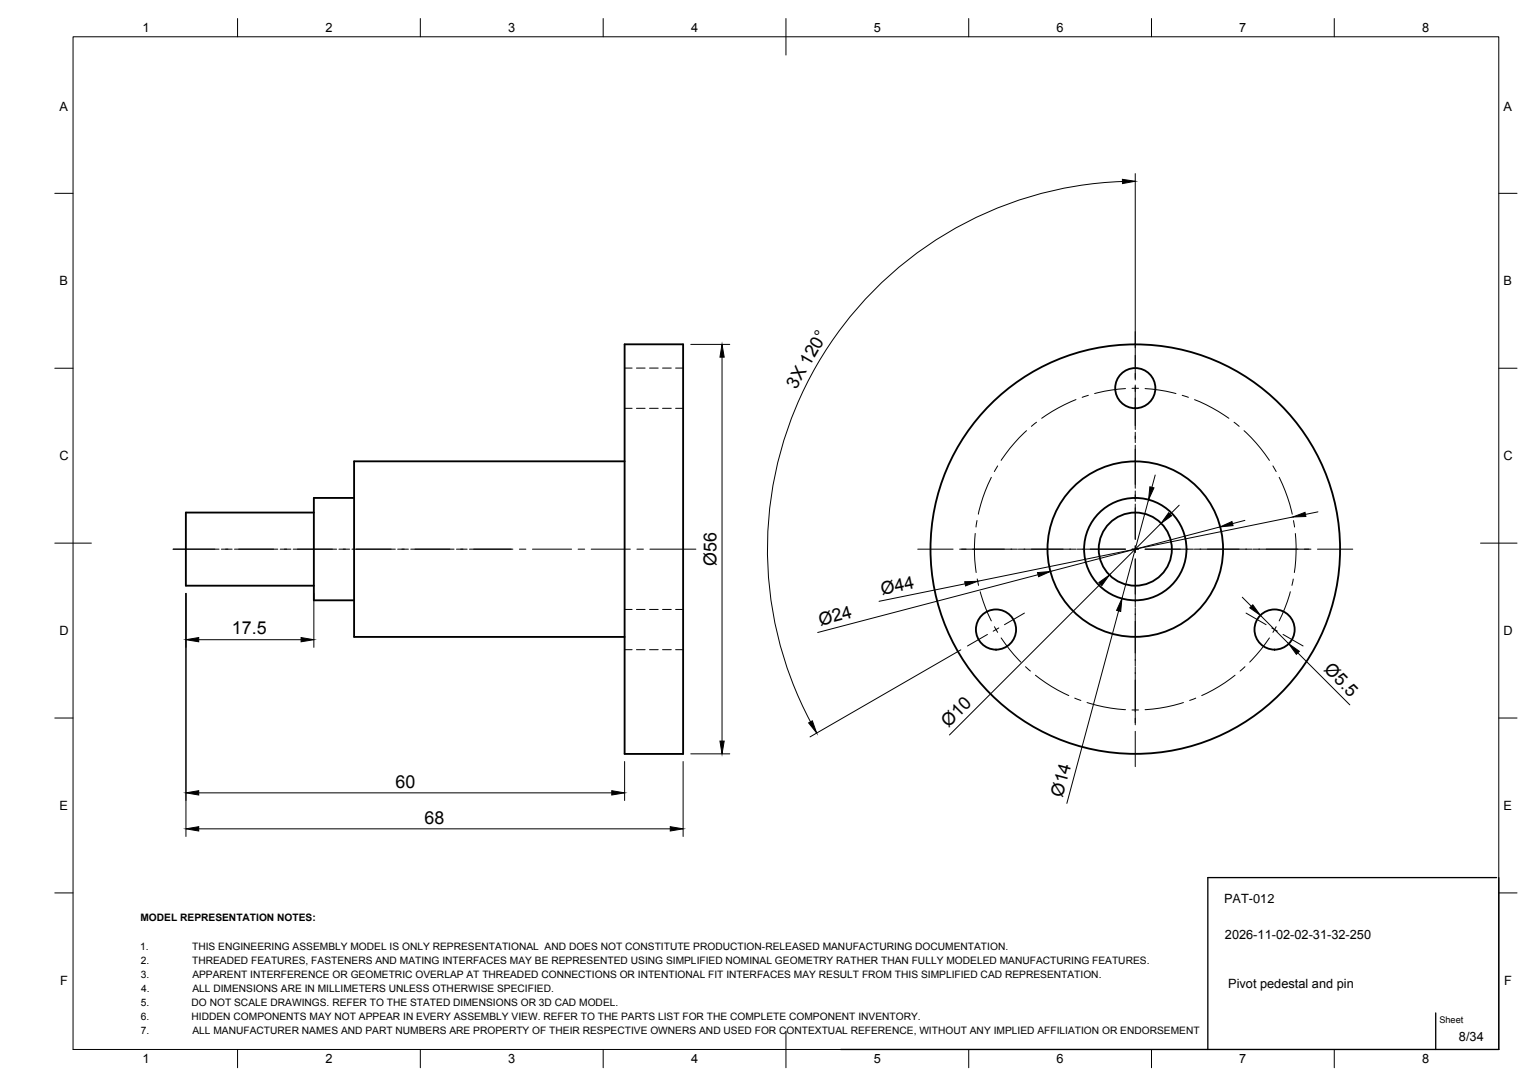
ISO-10303-21;
HEADER;
/* Generated by software containing ST-Developer
 * from STEP Tools, Inc. (www.steptools.com) 
 */

FILE_DESCRIPTION(
/* description */ ('Belt tensioner idler arm'),
/* implementation_level */ '2;1');

FILE_NAME(
/* name */ 'Pivot pedestal and pin.step',
/* time_stamp */ '2026-10-28T03:22:15-07:00',
/* author */ (''),
/* organization */ (''),
/* preprocessor_version */ 'ST-DEVELOPER v20.2',
/* originating_system */ 'Autodesk Translation Framework v15.17.0.0',
/* authorisation */ '');

FILE_SCHEMA (('AUTOMOTIVE_DESIGN { 1 0 10303 214 3 1 1 }'));
ENDSEC;

DATA;
#10=MECHANICAL_DESIGN_GEOMETRIC_PRESENTATION_REPRESENTATION('',(#450),#12779);
#382=SHAPE_REPRESENTATION_RELATIONSHIP('SRR','None',#12928,#416);
#416=ADVANCED_BREP_SHAPE_REPRESENTATION('',(#492),#12745);
#450=STYLED_ITEM('',(#13184),#492);
#492=MANIFOLD_SOLID_BREP('Body1',#6184);
#537=FACE_BOUND('',#1241,.T.);
#538=FACE_BOUND('',#1246,.T.);
#539=FACE_BOUND('',#1247,.T.);
#540=FACE_BOUND('',#1248,.T.);
#541=FACE_BOUND('',#1249,.T.);
#542=FACE_BOUND('',#1253,.T.);
#543=FACE_BOUND('',#1255,.T.);
#544=FACE_BOUND('',#1256,.T.);
#545=FACE_BOUND('',#1257,.T.);
#681=PLANE('',#6650);
#682=PLANE('',#6657);
#683=PLANE('',#6658);
#684=PLANE('',#6665);
#685=PLANE('',#6666);
#860=FACE_OUTER_BOUND('',#1237,.T.);
#861=FACE_OUTER_BOUND('',#1238,.T.);
#862=FACE_OUTER_BOUND('',#1239,.T.);
#863=FACE_OUTER_BOUND('',#1240,.T.);
#864=FACE_OUTER_BOUND('',#1242,.T.);
#865=FACE_OUTER_BOUND('',#1243,.T.);
#866=FACE_OUTER_BOUND('',#1244,.T.);
#867=FACE_OUTER_BOUND('',#1245,.T.);
#868=FACE_OUTER_BOUND('',#1250,.T.);
#869=FACE_OUTER_BOUND('',#1251,.T.);
#870=FACE_OUTER_BOUND('',#1252,.T.);
#871=FACE_OUTER_BOUND('',#1254,.T.);
#1237=EDGE_LOOP('',(#4188,#4189,#4190,#4191));
#1238=EDGE_LOOP('',(#4192,#4193,#4194,#4195));
#1239=EDGE_LOOP('',(#4196,#4197,#4198,#4199));
#1240=EDGE_LOOP('',(#4200));
#1241=EDGE_LOOP('',(#4201));
#1242=EDGE_LOOP('',(#4202,#4203,#4204,#4205));
#1243=EDGE_LOOP('',(#4206,#4207,#4208,#4209));
#1244=EDGE_LOOP('',(#4210));
#1245=EDGE_LOOP('',(#4211));
#1246=EDGE_LOOP('',(#4212));
#1247=EDGE_LOOP('',(#4213));
#1248=EDGE_LOOP('',(#4214));
#1249=EDGE_LOOP('',(#4215));
#1250=EDGE_LOOP('',(#4216,#4217,#4218,#4219));
#1251=EDGE_LOOP('',(#4220,#4221,#4222,#4223));
#1252=EDGE_LOOP('',(#4224));
#1253=EDGE_LOOP('',(#4225));
#1254=EDGE_LOOP('',(#4226));
#1255=EDGE_LOOP('',(#4227));
#1256=EDGE_LOOP('',(#4228));
#1257=EDGE_LOOP('',(#4229));
#1748=LINE('',#9562,#2097);
#1749=LINE('',#9568,#2098);
#1750=LINE('',#9574,#2099);
#1751=LINE('',#9583,#2100);
#1752=LINE('',#9588,#2101);
#1753=LINE('',#9597,#2102);
#1754=LINE('',#9602,#2103);
#2097=VECTOR('',#7556,0.275);
#2098=VECTOR('',#7563,0.275);
#2099=VECTOR('',#7570,0.275);
#2100=VECTOR('',#7581,0.7);
#2101=VECTOR('',#7588,0.5);
#2102=VECTOR('',#7599,2.8);
#2103=VECTOR('',#7606,1.2);
#2415=CIRCLE('',#6642,0.275);
#2416=CIRCLE('',#6643,0.275);
#2417=CIRCLE('',#6645,0.275);
#2418=CIRCLE('',#6646,0.275);
#2419=CIRCLE('',#6648,0.275);
#2420=CIRCLE('',#6649,0.275);
#2421=CIRCLE('',#6651,0.7);
#2422=CIRCLE('',#6652,0.5);
#2423=CIRCLE('',#6654,0.7);
#2424=CIRCLE('',#6656,0.5);
#2425=CIRCLE('',#6659,2.8);
#2426=CIRCLE('',#6660,1.2);
#2427=CIRCLE('',#6662,2.8);
#2428=CIRCLE('',#6664,1.2);
#2803=VERTEX_POINT('',#9559);
#2804=VERTEX_POINT('',#9561);
#2805=VERTEX_POINT('',#9565);
#2806=VERTEX_POINT('',#9567);
#2807=VERTEX_POINT('',#9571);
#2808=VERTEX_POINT('',#9573);
#2809=VERTEX_POINT('',#9577);
#2810=VERTEX_POINT('',#9579);
#2811=VERTEX_POINT('',#9582);
#2812=VERTEX_POINT('',#9586);
#2813=VERTEX_POINT('',#9591);
#2814=VERTEX_POINT('',#9593);
#2815=VERTEX_POINT('',#9596);
#2816=VERTEX_POINT('',#9600);
#3349=EDGE_CURVE('',#2803,#2803,#2415,.T.);
#3350=EDGE_CURVE('',#2803,#2804,#1748,.T.);
#3351=EDGE_CURVE('',#2804,#2804,#2416,.T.);
#3352=EDGE_CURVE('',#2805,#2805,#2417,.T.);
#3353=EDGE_CURVE('',#2805,#2806,#1749,.T.);
#3354=EDGE_CURVE('',#2806,#2806,#2418,.T.);
#3355=EDGE_CURVE('',#2807,#2807,#2419,.T.);
#3356=EDGE_CURVE('',#2807,#2808,#1750,.T.);
#3357=EDGE_CURVE('',#2808,#2808,#2420,.T.);
#3358=EDGE_CURVE('',#2809,#2809,#2421,.T.);
#3359=EDGE_CURVE('',#2810,#2810,#2422,.T.);
#3360=EDGE_CURVE('',#2809,#2811,#1751,.T.);
#3361=EDGE_CURVE('',#2811,#2811,#2423,.T.);
#3362=EDGE_CURVE('',#2812,#2812,#2424,.T.);
#3363=EDGE_CURVE('',#2812,#2810,#1752,.T.);
#3364=EDGE_CURVE('',#2813,#2813,#2425,.T.);
#3365=EDGE_CURVE('',#2814,#2814,#2426,.T.);
#3366=EDGE_CURVE('',#2813,#2815,#1753,.T.);
#3367=EDGE_CURVE('',#2815,#2815,#2427,.T.);
#3368=EDGE_CURVE('',#2816,#2816,#2428,.T.);
#3369=EDGE_CURVE('',#2816,#2814,#1754,.T.);
#4188=ORIENTED_EDGE('',*,*,#3349,.F.);
#4189=ORIENTED_EDGE('',*,*,#3350,.T.);
#4190=ORIENTED_EDGE('',*,*,#3351,.F.);
#4191=ORIENTED_EDGE('',*,*,#3350,.F.);
#4192=ORIENTED_EDGE('',*,*,#3352,.F.);
#4193=ORIENTED_EDGE('',*,*,#3353,.T.);
#4194=ORIENTED_EDGE('',*,*,#3354,.F.);
#4195=ORIENTED_EDGE('',*,*,#3353,.F.);
#4196=ORIENTED_EDGE('',*,*,#3355,.F.);
#4197=ORIENTED_EDGE('',*,*,#3356,.T.);
#4198=ORIENTED_EDGE('',*,*,#3357,.F.);
#4199=ORIENTED_EDGE('',*,*,#3356,.F.);
#4200=ORIENTED_EDGE('',*,*,#3358,.T.);
#4201=ORIENTED_EDGE('',*,*,#3359,.F.);
#4202=ORIENTED_EDGE('',*,*,#3358,.F.);
#4203=ORIENTED_EDGE('',*,*,#3360,.T.);
#4204=ORIENTED_EDGE('',*,*,#3361,.F.);
#4205=ORIENTED_EDGE('',*,*,#3360,.F.);
#4206=ORIENTED_EDGE('',*,*,#3362,.F.);
#4207=ORIENTED_EDGE('',*,*,#3363,.T.);
#4208=ORIENTED_EDGE('',*,*,#3359,.T.);
#4209=ORIENTED_EDGE('',*,*,#3363,.F.);
#4210=ORIENTED_EDGE('',*,*,#3362,.T.);
#4211=ORIENTED_EDGE('',*,*,#3364,.T.);
#4212=ORIENTED_EDGE('',*,*,#3351,.T.);
#4213=ORIENTED_EDGE('',*,*,#3354,.T.);
#4214=ORIENTED_EDGE('',*,*,#3357,.T.);
#4215=ORIENTED_EDGE('',*,*,#3365,.F.);
#4216=ORIENTED_EDGE('',*,*,#3364,.F.);
#4217=ORIENTED_EDGE('',*,*,#3366,.T.);
#4218=ORIENTED_EDGE('',*,*,#3367,.T.);
#4219=ORIENTED_EDGE('',*,*,#3366,.F.);
#4220=ORIENTED_EDGE('',*,*,#3368,.F.);
#4221=ORIENTED_EDGE('',*,*,#3369,.T.);
#4222=ORIENTED_EDGE('',*,*,#3365,.T.);
#4223=ORIENTED_EDGE('',*,*,#3369,.F.);
#4224=ORIENTED_EDGE('',*,*,#3368,.T.);
#4225=ORIENTED_EDGE('',*,*,#3361,.T.);
#4226=ORIENTED_EDGE('',*,*,#3367,.F.);
#4227=ORIENTED_EDGE('',*,*,#3349,.T.);
#4228=ORIENTED_EDGE('',*,*,#3352,.T.);
#4229=ORIENTED_EDGE('',*,*,#3355,.T.);
#5667=CYLINDRICAL_SURFACE('',#6641,0.275);
#5668=CYLINDRICAL_SURFACE('',#6644,0.275);
#5669=CYLINDRICAL_SURFACE('',#6647,0.275);
#5670=CYLINDRICAL_SURFACE('',#6653,0.7);
#5671=CYLINDRICAL_SURFACE('',#6655,0.5);
#5672=CYLINDRICAL_SURFACE('',#6661,2.8);
#5673=CYLINDRICAL_SURFACE('',#6663,1.2);
#5837=ADVANCED_FACE('',(#860),#5667,.F.);
#5838=ADVANCED_FACE('',(#861),#5668,.F.);
#5839=ADVANCED_FACE('',(#862),#5669,.F.);
#5840=ADVANCED_FACE('',(#863,#537),#681,.T.);
#5841=ADVANCED_FACE('',(#864),#5670,.T.);
#5842=ADVANCED_FACE('',(#865),#5671,.T.);
#5843=ADVANCED_FACE('',(#866),#682,.T.);
#5844=ADVANCED_FACE('',(#867,#538,#539,#540,#541),#683,.T.);
#5845=ADVANCED_FACE('',(#868),#5672,.T.);
#5846=ADVANCED_FACE('',(#869),#5673,.T.);
#5847=ADVANCED_FACE('',(#870,#542),#684,.T.);
#5848=ADVANCED_FACE('',(#871,#543,#544,#545),#685,.F.);
#6184=CLOSED_SHELL('',(#5837,#5838,#5839,#5840,#5841,#5842,#5843,#5844,
#5845,#5846,#5847,#5848));
#6640=AXIS2_PLACEMENT_3D('',#9557,#7550,#7551);
#6641=AXIS2_PLACEMENT_3D('',#9558,#7552,#7553);
#6642=AXIS2_PLACEMENT_3D('',#9560,#7554,#7555);
#6643=AXIS2_PLACEMENT_3D('',#9563,#7557,#7558);
#6644=AXIS2_PLACEMENT_3D('',#9564,#7559,#7560);
#6645=AXIS2_PLACEMENT_3D('',#9566,#7561,#7562);
#6646=AXIS2_PLACEMENT_3D('',#9569,#7564,#7565);
#6647=AXIS2_PLACEMENT_3D('',#9570,#7566,#7567);
#6648=AXIS2_PLACEMENT_3D('',#9572,#7568,#7569);
#6649=AXIS2_PLACEMENT_3D('',#9575,#7571,#7572);
#6650=AXIS2_PLACEMENT_3D('',#9576,#7573,#7574);
#6651=AXIS2_PLACEMENT_3D('',#9578,#7575,#7576);
#6652=AXIS2_PLACEMENT_3D('',#9580,#7577,#7578);
#6653=AXIS2_PLACEMENT_3D('',#9581,#7579,#7580);
#6654=AXIS2_PLACEMENT_3D('',#9584,#7582,#7583);
#6655=AXIS2_PLACEMENT_3D('',#9585,#7584,#7585);
#6656=AXIS2_PLACEMENT_3D('',#9587,#7586,#7587);
#6657=AXIS2_PLACEMENT_3D('',#9589,#7589,#7590);
#6658=AXIS2_PLACEMENT_3D('',#9590,#7591,#7592);
#6659=AXIS2_PLACEMENT_3D('',#9592,#7593,#7594);
#6660=AXIS2_PLACEMENT_3D('',#9594,#7595,#7596);
#6661=AXIS2_PLACEMENT_3D('',#9595,#7597,#7598);
#6662=AXIS2_PLACEMENT_3D('',#9598,#7600,#7601);
#6663=AXIS2_PLACEMENT_3D('',#9599,#7602,#7603);
#6664=AXIS2_PLACEMENT_3D('',#9601,#7604,#7605);
#6665=AXIS2_PLACEMENT_3D('',#9603,#7607,#7608);
#6666=AXIS2_PLACEMENT_3D('',#9604,#7609,#7610);
#7550=DIRECTION('axis',(0.,0.,1.));
#7551=DIRECTION('refdir',(1.,0.,0.));
#7552=DIRECTION('center_axis',(0.,0.,1.));
#7553=DIRECTION('ref_axis',(1.,0.,0.));
#7554=DIRECTION('center_axis',(0.,0.,1.));
#7555=DIRECTION('ref_axis',(1.,0.,0.));
#7556=DIRECTION('',(0.,0.,1.));
#7557=DIRECTION('center_axis',(0.,0.,-1.));
#7558=DIRECTION('ref_axis',(1.,0.,0.));
#7559=DIRECTION('center_axis',(0.,0.,1.));
#7560=DIRECTION('ref_axis',(1.,0.,0.));
#7561=DIRECTION('center_axis',(0.,0.,1.));
#7562=DIRECTION('ref_axis',(1.,0.,0.));
#7563=DIRECTION('',(0.,0.,1.));
#7564=DIRECTION('center_axis',(0.,0.,-1.));
#7565=DIRECTION('ref_axis',(1.,0.,0.));
#7566=DIRECTION('center_axis',(0.,0.,1.));
#7567=DIRECTION('ref_axis',(1.,0.,0.));
#7568=DIRECTION('center_axis',(0.,0.,1.));
#7569=DIRECTION('ref_axis',(1.,0.,0.));
#7570=DIRECTION('',(0.,0.,1.));
#7571=DIRECTION('center_axis',(0.,0.,-1.));
#7572=DIRECTION('ref_axis',(1.,0.,0.));
#7573=DIRECTION('center_axis',(0.,0.,1.));
#7574=DIRECTION('ref_axis',(1.,0.,0.));
#7575=DIRECTION('center_axis',(0.,0.,1.));
#7576=DIRECTION('ref_axis',(1.,0.,0.));
#7577=DIRECTION('center_axis',(0.,0.,1.));
#7578=DIRECTION('ref_axis',(1.,0.,0.));
#7579=DIRECTION('center_axis',(0.,0.,1.));
#7580=DIRECTION('ref_axis',(1.,0.,0.));
#7581=DIRECTION('',(0.,0.,-1.));
#7582=DIRECTION('center_axis',(0.,0.,-1.));
#7583=DIRECTION('ref_axis',(1.,0.,0.));
#7584=DIRECTION('center_axis',(0.,0.,1.));
#7585=DIRECTION('ref_axis',(1.,0.,0.));
#7586=DIRECTION('center_axis',(0.,0.,1.));
#7587=DIRECTION('ref_axis',(1.,0.,0.));
#7588=DIRECTION('',(0.,0.,-1.));
#7589=DIRECTION('center_axis',(0.,0.,1.));
#7590=DIRECTION('ref_axis',(1.,0.,0.));
#7591=DIRECTION('center_axis',(0.,0.,1.));
#7592=DIRECTION('ref_axis',(1.,0.,0.));
#7593=DIRECTION('center_axis',(0.,0.,1.));
#7594=DIRECTION('ref_axis',(1.,0.,0.));
#7595=DIRECTION('center_axis',(0.,0.,1.));
#7596=DIRECTION('ref_axis',(1.,0.,0.));
#7597=DIRECTION('center_axis',(0.,0.,1.));
#7598=DIRECTION('ref_axis',(1.,0.,0.));
#7599=DIRECTION('',(0.,0.,-1.));
#7600=DIRECTION('center_axis',(0.,0.,1.));
#7601=DIRECTION('ref_axis',(1.,0.,0.));
#7602=DIRECTION('center_axis',(0.,0.,1.));
#7603=DIRECTION('ref_axis',(1.,0.,0.));
#7604=DIRECTION('center_axis',(0.,0.,1.));
#7605=DIRECTION('ref_axis',(1.,0.,0.));
#7606=DIRECTION('',(0.,0.,-1.));
#7607=DIRECTION('center_axis',(0.,0.,1.));
#7608=DIRECTION('ref_axis',(1.,0.,0.));
#7609=DIRECTION('center_axis',(0.,0.,1.));
#7610=DIRECTION('ref_axis',(1.,0.,0.));
#9557=CARTESIAN_POINT('',(0.,0.,0.));
#9558=CARTESIAN_POINT('Origin',(2.2,0.,-0.1));
#9559=CARTESIAN_POINT('',(1.925,-3.36777869765522E-17,0.));
#9560=CARTESIAN_POINT('Origin',(2.2,0.,0.));
#9561=CARTESIAN_POINT('',(1.925,3.36777869765522E-17,0.8));
#9562=CARTESIAN_POINT('',(1.925,-3.36777869765522E-17,-0.1));
#9563=CARTESIAN_POINT('Origin',(2.2,0.,0.8));
#9564=CARTESIAN_POINT('Origin',(-1.1,1.90525588832577,-0.1));
#9565=CARTESIAN_POINT('',(-1.375,1.90525588832577,0.));
#9566=CARTESIAN_POINT('Origin',(-1.1,1.90525588832577,0.));
#9567=CARTESIAN_POINT('',(-1.375,1.90525588832577,0.8));
#9568=CARTESIAN_POINT('',(-1.375,1.90525588832577,-0.1));
#9569=CARTESIAN_POINT('Origin',(-1.1,1.90525588832577,0.8));
#9570=CARTESIAN_POINT('Origin',(-1.1,-1.90525588832576,-0.1));
#9571=CARTESIAN_POINT('',(-1.375,-1.90525588832576,0.));
#9572=CARTESIAN_POINT('Origin',(-1.1,-1.90525588832576,0.));
#9573=CARTESIAN_POINT('',(-1.375,-1.90525588832576,0.8));
#9574=CARTESIAN_POINT('',(-1.375,-1.90525588832576,-0.1));
#9575=CARTESIAN_POINT('Origin',(-1.1,-1.90525588832576,0.8));
#9576=CARTESIAN_POINT('Origin',(0.,0.,5.05));
#9577=CARTESIAN_POINT('',(-0.7,-8.57252759403147E-17,5.05));
#9578=CARTESIAN_POINT('Origin',(0.,0.,5.05));
#9579=CARTESIAN_POINT('',(-0.5,-6.12323399573677E-17,5.05));
#9580=CARTESIAN_POINT('Origin',(0.,0.,5.05));
#9581=CARTESIAN_POINT('Origin',(0.,0.,4.5));
#9582=CARTESIAN_POINT('',(-0.7,-8.57252759403147E-17,4.5));
#9583=CARTESIAN_POINT('',(-0.7,-8.57252759403147E-17,4.5));
#9584=CARTESIAN_POINT('Origin',(0.,0.,4.5));
#9585=CARTESIAN_POINT('Origin',(0.,0.,4.5));
#9586=CARTESIAN_POINT('',(-0.5,-6.12323399573677E-17,6.8));
#9587=CARTESIAN_POINT('Origin',(0.,0.,6.8));
#9588=CARTESIAN_POINT('',(-0.5,-6.12323399573677E-17,4.5));
#9589=CARTESIAN_POINT('Origin',(0.,0.,6.8));
#9590=CARTESIAN_POINT('Origin',(0.,0.,0.8));
#9591=CARTESIAN_POINT('',(-2.8,-3.42901103761259E-16,0.8));
#9592=CARTESIAN_POINT('Origin',(0.,0.,0.8));
#9593=CARTESIAN_POINT('',(-1.2,-1.46957615897682E-16,0.8));
#9594=CARTESIAN_POINT('Origin',(0.,0.,0.8));
#9595=CARTESIAN_POINT('Origin',(0.,0.,0.));
#9596=CARTESIAN_POINT('',(-2.8,-3.42901103761259E-16,0.));
#9597=CARTESIAN_POINT('',(-2.8,-3.42901103761259E-16,0.));
#9598=CARTESIAN_POINT('Origin',(0.,0.,0.));
#9599=CARTESIAN_POINT('Origin',(0.,0.,0.));
#9600=CARTESIAN_POINT('',(-1.2,-1.46957615897682E-16,4.5));
#9601=CARTESIAN_POINT('Origin',(0.,0.,4.5));
#9602=CARTESIAN_POINT('',(-1.2,-1.46957615897682E-16,0.));
#9603=CARTESIAN_POINT('Origin',(0.,0.,4.5));
#9604=CARTESIAN_POINT('Origin',(0.,0.,0.));
#12705=UNCERTAINTY_MEASURE_WITH_UNIT(LENGTH_MEASURE(0.001),#12780,
'DISTANCE_ACCURACY_VALUE',
'Maximum model space distance between geometric entities at asserted c
onnectivities');
#12739=UNCERTAINTY_MEASURE_WITH_UNIT(LENGTH_MEASURE(0.001),#12780,
'DISTANCE_ACCURACY_VALUE',
'Maximum model space distance between geometric entities at asserted c
onnectivities');
#12745=(
GEOMETRIC_REPRESENTATION_CONTEXT(3)
GLOBAL_UNCERTAINTY_ASSIGNED_CONTEXT((#12705))
GLOBAL_UNIT_ASSIGNED_CONTEXT((#12780,#12782,#12783))
REPRESENTATION_CONTEXT('','3D')
);
#12779=(
GEOMETRIC_REPRESENTATION_CONTEXT(3)
GLOBAL_UNCERTAINTY_ASSIGNED_CONTEXT((#12739))
GLOBAL_UNIT_ASSIGNED_CONTEXT((#12780,#12782,#12783))
REPRESENTATION_CONTEXT('','3D')
);
#12780=(
LENGTH_UNIT()
NAMED_UNIT(*)
SI_UNIT(.CENTI.,.METRE.)
);
#12782=(
NAMED_UNIT(*)
PLANE_ANGLE_UNIT()
SI_UNIT($,.RADIAN.)
);
#12783=(
NAMED_UNIT(*)
SI_UNIT($,.STERADIAN.)
SOLID_ANGLE_UNIT()
);
#12789=SHAPE_DEFINITION_REPRESENTATION(#12828,#12928);
#12828=PRODUCT_DEFINITION_SHAPE('',$,#12968);
#12928=SHAPE_REPRESENTATION('',(#6640),#12745);
#12962=PRODUCT_DEFINITION_CONTEXT('part definition',#13081,'design');
#12968=PRODUCT_DEFINITION('Pivot pedestal and pin',
'Pivot pedestal and pin',#13007,#12962);
#13007=PRODUCT_DEFINITION_FORMATION('',$,#13088);
#13081=APPLICATION_CONTEXT(
'Core Data for Automotive Mechanical Design Process');
#13082=PRODUCT_CONTEXT('part definition',#13081,'mechanical');
#13088=PRODUCT('Pivot pedestal and pin','Pivot pedestal and pin',
'Pivot pedestal and pin',(#13082));
#13178=COLOUR_RGB('Grey',0.48,0.52,0.57);
#13179=FILL_AREA_STYLE_COLOUR('',#13178);
#13180=FILL_AREA_STYLE('',(#13179));
#13181=SURFACE_STYLE_FILL_AREA(#13180);
#13182=SURFACE_SIDE_STYLE('',(#13181));
#13183=SURFACE_STYLE_USAGE(.BOTH.,#13182);
#13184=PRESENTATION_STYLE_ASSIGNMENT((#13183));
ENDSEC;
END-ISO-10303-21;
